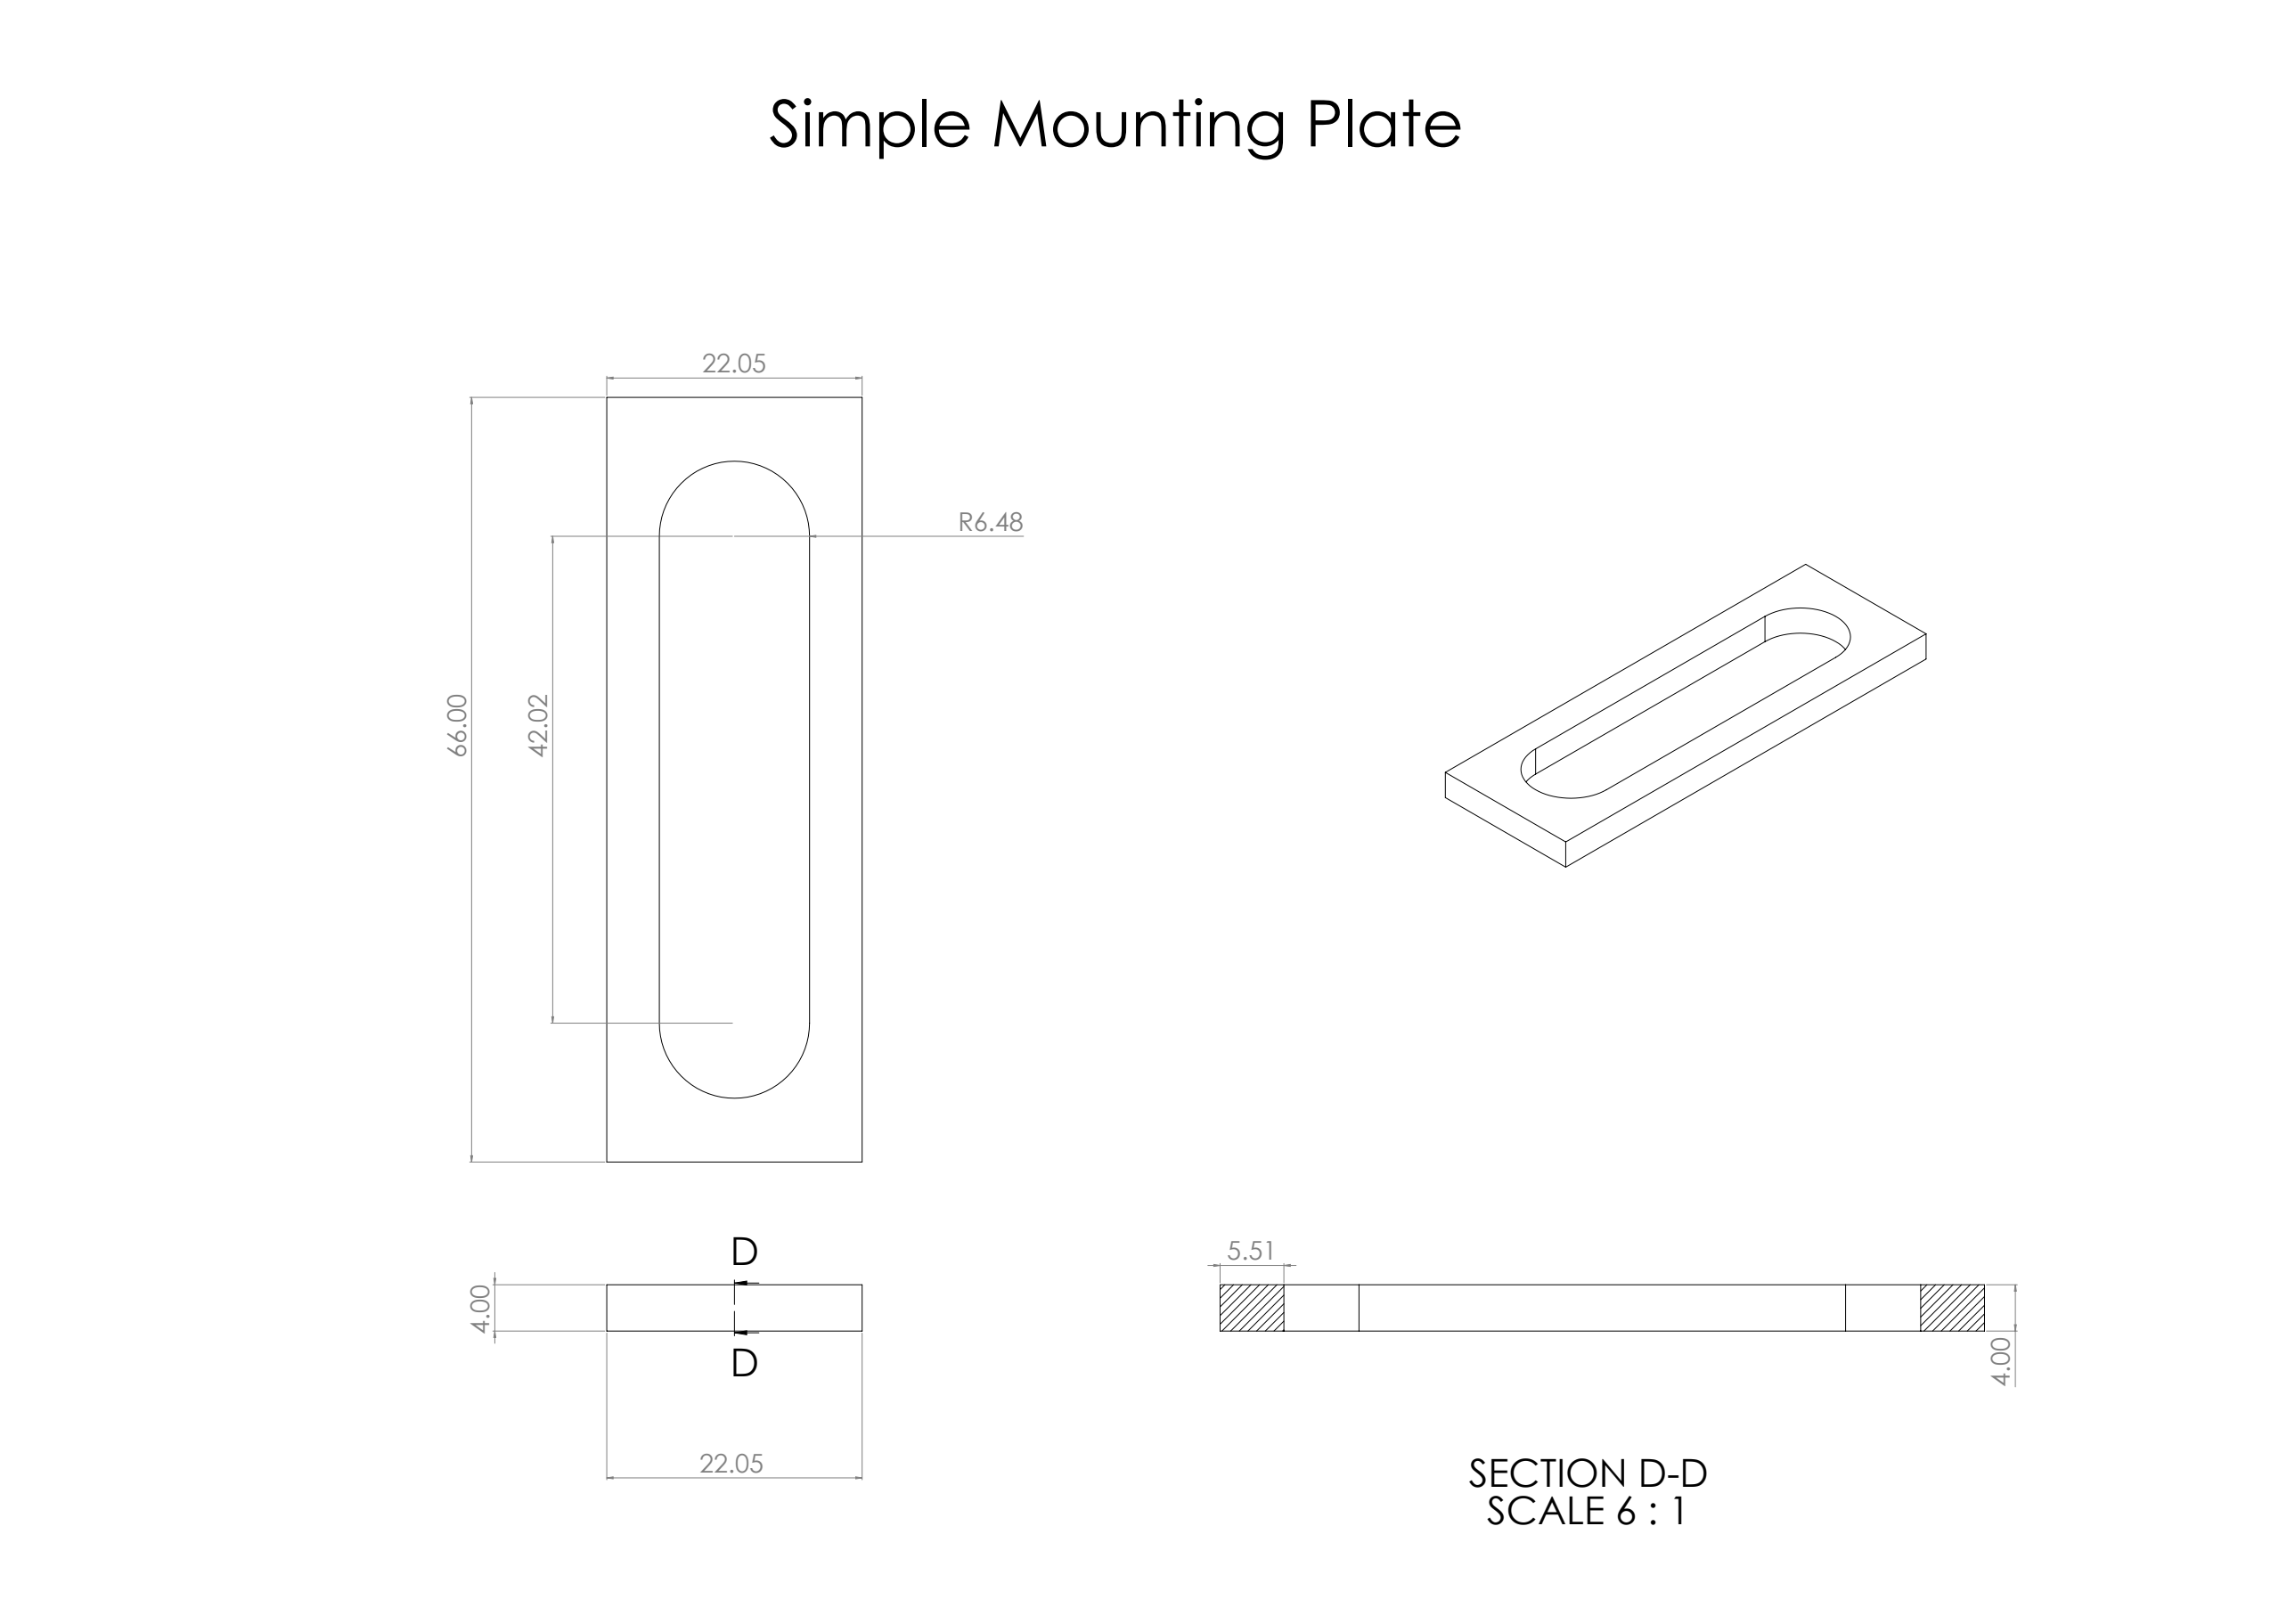
ISO-10303-21;
HEADER;
FILE_DESCRIPTION (('STEP AP214'),
    '1' );
FILE_NAME ('Simple Mounting Plate.step',
    '2026-10-24T21:31:31',
    ( '' ),
    ( '' ),
    'SwSTEP 2.0',
    'SolidWorks 2025',
    '' );
FILE_SCHEMA (( 'AUTOMOTIVE_DESIGN' ));
ENDSEC;

DATA;
#29=DIRECTION ( 'NONE',  ( 1.000000000000000000, 0.000000000000000000, 0.000000000000000000 ) ) ;
#109=DIRECTION ( 'NONE',  ( 0.000000000000000000, 1.000000000000000000, 0.000000000000000000 ) ) ;
#168=( NAMED_UNIT ( * ) PLANE_ANGLE_UNIT ( ) SI_UNIT ( $, .RADIAN. ) );
#183=CIRCLE ( 'NONE', #7797, 6.484807146443463566 ) ;
#379=LINE ( 'NONE', #14467, #12326 ) ;
#390=FACE_OUTER_BOUND ( 'NONE', #10750, .T. ) ;
#422=ORIENTED_EDGE ( 'NONE', *, *, #2866, .F. ) ;
#457=CARTESIAN_POINT ( 'NONE',  ( 80.18290120114222930, 29.52935533987996664, -21.00807340887166674 ) ) ;
#476=EDGE_CURVE ( 'NONE', #7436, #10628, #11850, .T. ) ;
#568=CIRCLE ( 'NONE', #806, 6.484807146443463566 ) ;
#583=FACE_OUTER_BOUND ( 'NONE', #10613, .T. ) ;
#609=EDGE_CURVE ( 'NONE', #7436, #1277, #1384, .T. ) ;
#623=( LENGTH_UNIT ( ) NAMED_UNIT ( * ) SI_UNIT ( .MILLI., .METRE. ) );
#791=VERTEX_POINT ( 'NONE', #9257 ) ;
#806=AXIS2_PLACEMENT_3D ( 'NONE', #12943, #2078, #13935 ) ;
#820=EDGE_LOOP ( 'NONE', ( #5722, #8057, #10459, #9791, #8309 ) ) ;
#827=CARTESIAN_POINT ( 'NONE',  ( 80.18290120114222930, 29.52935533987996664, 21.00807340887166674 ) ) ;
#863=CARTESIAN_POINT ( 'NONE',  ( 67.21328690825529861, 29.52935533987996664, -21.00807340887166674 ) ) ;
#928=AXIS2_PLACEMENT_3D ( 'NONE', #14541, #7614, #1981 ) ;
#984=DIRECTION ( 'NONE',  ( 0.000000000000000000, 0.000000000000000000, 1.000000000000000000 ) ) ;
#1030=AXIS2_PLACEMENT_3D ( 'NONE', #11882, #5895, #6042 ) ;
#1049=ORIENTED_EDGE ( 'NONE', *, *, #13035, .F. ) ;
#1079=DIRECTION ( 'NONE',  ( 0.000000000000000000, 0.000000000000000000, 1.000000000000000000 ) ) ;
#1080=ORIENTED_EDGE ( 'NONE', *, *, #1195, .F. ) ;
#1195=EDGE_CURVE ( 'NONE', #10628, #10836, #7216, .T. ) ;
#1277=VERTEX_POINT ( 'NONE', #3964 ) ;
#1327=AXIS2_PLACEMENT_3D ( 'NONE', #8905, #1894, #6592 ) ;
#1376=LINE ( 'NONE', #7228, #11447 ) ;
#1384=LINE ( 'NONE', #457, #2184 ) ;
#1482=CARTESIAN_POINT ( 'NONE',  ( 0.000000000000000000, 25.52935533987996664, 0.000000000000000000 ) ) ;
#1489=ORIENTED_EDGE ( 'NONE', *, *, #10313, .T. ) ;
#1494=DIRECTION ( 'NONE',  ( 0.000000000000000000, 0.000000000000000000, 1.000000000000000000 ) ) ;
#1505=UNCERTAINTY_MEASURE_WITH_UNIT (LENGTH_MEASURE( 1.000000000000000082E-05 ), #623, 'distance_accuracy_value', 'NONE');
#1520=DIRECTION ( 'NONE',  ( -0.000000000000000000, -0.000000000000000000, -1.000000000000000000 ) ) ;
#1550=ORIENTED_EDGE ( 'NONE', *, *, #14612, .F. ) ;
#1557=SHAPE_REPRESENTATION ( 'Simple Mounting Plate', ( #6315 ), #10740 ) ;
#1651=UNCERTAINTY_MEASURE_WITH_UNIT (LENGTH_MEASURE( 1.000000000000000082E-05 ), #7097, 'distance_accuracy_value', 'NONE');
#1684=DIRECTION ( 'NONE',  ( -1.000000000000000000, -0.000000000000000000, -0.000000000000000000 ) ) ;
#1734=DIRECTION ( 'NONE',  ( 1.000000000000000000, 0.000000000000000000, 0.000000000000000000 ) ) ;
#1764=VECTOR ( 'NONE', #15120, 1000.000000000000000 ) ;
#1873=ADVANCED_FACE ( 'NONE', ( #10648, #14344 ), #12017, .F. ) ;
#1894=DIRECTION ( 'NONE',  ( -1.000000000000000000, 0.000000000000000000, 0.000000000000000000 ) ) ;
#1912=ORIENTED_EDGE ( 'NONE', *, *, #2866, .T. ) ;
#1981=DIRECTION ( 'NONE',  ( 0.000000000000000000, 0.000000000000000000, -1.000000000000000000 ) ) ;
#2036=EDGE_CURVE ( 'NONE', #12382, #4409, #3728, .T. ) ;
#2078=DIRECTION ( 'NONE',  ( 0.000000000000000000, 1.000000000000000000, 0.000000000000000000 ) ) ;
#2087=SHAPE_REPRESENTATION_RELATIONSHIP ( 'NONE' , 'NONE' ,  #1557, #14388 ) ;
#2104=CYLINDRICAL_SURFACE ( 'NONE', #3264, 6.484807146443463566 ) ;
#2154=CLOSED_SHELL ( 'NONE', ( #8223, #12212, #1873, #6816, #3020, #5563, #3592, #7389, #14535, #15006, #9629 ) ) ;
#2184=VECTOR ( 'NONE', #14243, 1000.000000000000000 ) ;
#2233=DIRECTION ( 'NONE',  ( -0.000000000000000000, -1.000000000000000000, -0.000000000000000000 ) ) ;
#2372=ORIENTED_EDGE ( 'NONE', *, *, #14612, .T. ) ;
#2603=CARTESIAN_POINT ( 'NONE',  ( 62.67308791069655882, 25.52935533987996664, -33.00000000000013500 ) ) ;
#2662=ORIENTED_EDGE ( 'NONE', *, *, #6455, .F. ) ;
#2724=VECTOR ( 'NONE', #7198, 1000.000000000000000 ) ;
#2775=AXIS2_PLACEMENT_3D ( 'NONE', #14477, #3923, #8618 ) ;
#2819=PLANE ( 'NONE',  #15180 ) ;
#2866=EDGE_CURVE ( 'NONE', #3904, #14153, #13128, .T. ) ;
#2949=CARTESIAN_POINT ( 'NONE',  ( 73.69809405469877106, 29.52935533987996664, -21.00807340887166674 ) ) ;
#2992=ORIENTED_EDGE ( 'NONE', *, *, #10935, .F. ) ;
#3020=ADVANCED_FACE ( 'NONE', ( #5114 ), #11033, .F. ) ;
#3026=CARTESIAN_POINT ( 'NONE',  ( 80.18290120114222930, 25.52935533987996664, 21.00807340887166674 ) ) ;
#3032=DIRECTION ( 'NONE',  ( 0.000000000000000000, 0.000000000000000000, -1.000000000000000000 ) ) ;
#3108=CARTESIAN_POINT ( 'NONE',  ( 62.67308791069655882, 29.52935533987996664, 33.00000000000014211 ) ) ;
#3186=DIRECTION ( 'NONE',  ( 0.000000000000000000, 0.000000000000000000, 1.000000000000000000 ) ) ;
#3189=EDGE_CURVE ( 'NONE', #14936, #3904, #9655, .T. ) ;
#3207=FACE_OUTER_BOUND ( 'NONE', #4528, .T. ) ;
#3235=PLANE ( 'NONE',  #15227 ) ;
#3263=DIRECTION ( 'NONE',  ( -0.000000000000000000, -1.000000000000000000, -0.000000000000000000 ) ) ;
#3264=AXIS2_PLACEMENT_3D ( 'NONE', #6802, #13886, #3340 ) ;
#3284=ORIENTED_EDGE ( 'NONE', *, *, #5084, .F. ) ;
#3339=ORIENTED_EDGE ( 'NONE', *, *, #10313, .F. ) ;
#3340=DIRECTION ( 'NONE',  ( 0.000000000000000000, 0.000000000000000000, -1.000000000000000000 ) ) ;
#3384=FACE_OUTER_BOUND ( 'NONE', #10476, .T. ) ;
#3387=VECTOR ( 'NONE', #8666, 1000.000000000000000 ) ;
#3517=PRODUCT_DEFINITION_CONTEXT ( 'detailed design', #5959, 'design' ) ;
#3592=ADVANCED_FACE ( 'NONE', ( #10240 ), #3235, .F. ) ;
#3719=CARTESIAN_POINT ( 'NONE',  ( 84.72310019870096198, 29.52935533987996664, -33.00000000000013500 ) ) ;
#3728=LINE ( 'NONE', #14048, #4112 ) ;
#3738=VERTEX_POINT ( 'NONE', #6599 ) ;
#3748=CARTESIAN_POINT ( 'NONE',  ( 80.18290120114222930, 25.52935533987996664, -21.00807340887166674 ) ) ;
#3796=CARTESIAN_POINT ( 'NONE',  ( 80.18290120114222930, 29.52935533987996664, -21.00807340887166674 ) ) ;
#3904=VERTEX_POINT ( 'NONE', #5267 ) ;
#3923=DIRECTION ( 'NONE',  ( 1.000000000000000000, 0.000000000000000000, 0.000000000000000000 ) ) ;
#3946=DIRECTION ( 'NONE',  ( -1.000000000000000000, 0.000000000000000000, -0.000000000000000000 ) ) ;
#3964=CARTESIAN_POINT ( 'NONE',  ( 80.18290120114222930, 29.52935533987996664, -21.00807340887166674 ) ) ;
#3989=DIRECTION ( 'NONE',  ( -0.000000000000000000, -0.000000000000000000, -1.000000000000000000 ) ) ;
#4000=EDGE_CURVE ( 'NONE', #11210, #8448, #4643, .T. ) ;
#4022=ORIENTED_EDGE ( 'NONE', *, *, #7061, .T. ) ;
#4082=CARTESIAN_POINT ( 'NONE',  ( 0.000000000000000000, 0.000000000000000000, 0.000000000000000000 ) ) ;
#4112=VECTOR ( 'NONE', #10512, 1000.000000000000000 ) ;
#4123=ORIENTED_EDGE ( 'NONE', *, *, #5084, .T. ) ;
#4172=VERTEX_POINT ( 'NONE', #15048 ) ;
#4217=CIRCLE ( 'NONE', #1030, 6.484807146443463566 ) ;
#4250=VERTEX_POINT ( 'NONE', #6048 ) ;
#4296=CARTESIAN_POINT ( 'NONE',  ( 0.000000000000000000, 29.52935533987996664, 0.000000000000000000 ) ) ;
#4311=AXIS2_PLACEMENT_3D ( 'NONE', #4296, #4456, #8001 ) ;
#4409=VERTEX_POINT ( 'NONE', #7856 ) ;
#4443=VERTEX_POINT ( 'NONE', #10395 ) ;
#4456=DIRECTION ( 'NONE',  ( 0.000000000000000000, 1.000000000000000000, 0.000000000000000000 ) ) ;
#4528=EDGE_LOOP ( 'NONE', ( #11682, #1049, #9936, #1912 ) ) ;
#4547=EDGE_LOOP ( 'NONE', ( #14272, #13147, #6987, #3284 ) ) ;
#4643=LINE ( 'NONE', #863, #6660 ) ;
#4668=AXIS2_PLACEMENT_3D ( 'NONE', #14874, #3263, #5740 ) ;
#4759=VECTOR ( 'NONE', #3989, 1000.000000000000000 ) ;
#4773=DIRECTION ( 'NONE',  ( 0.000000000000000000, 0.000000000000000000, 1.000000000000000000 ) ) ;
#4825=AXIS2_PLACEMENT_3D ( 'NONE', #8741, #9919, #12290 ) ;
#4891=CARTESIAN_POINT ( 'NONE',  ( 84.72310019870096198, 29.52935533987996664, 33.00000000000014211 ) ) ;
#4982=VECTOR ( 'NONE', #12387, 1000.000000000000000 ) ;
#4984=CIRCLE ( 'NONE', #13574, 6.484807146443463566 ) ;
#4992=ORIENTED_EDGE ( 'NONE', *, *, #11137, .T. ) ;
#5036=CARTESIAN_POINT ( 'NONE',  ( 73.69809405469877106, 25.52935533987996664, -21.00807340887166674 ) ) ;
#5084=EDGE_CURVE ( 'NONE', #4409, #8448, #4984, .T. ) ;
#5086=PLANE ( 'NONE',  #2775 ) ;
#5114=FACE_OUTER_BOUND ( 'NONE', #5541, .T. ) ;
#5236=ORIENTED_EDGE ( 'NONE', *, *, #13202, .T. ) ;
#5267=CARTESIAN_POINT ( 'NONE',  ( 84.72310019870096198, 29.52935533987996664, 33.00000000000014211 ) ) ;
#5357=CARTESIAN_POINT ( 'NONE',  ( 67.21328690825529861, 29.52935533987996664, 21.00807340887166674 ) ) ;
#5366=PLANE ( 'NONE',  #4825 ) ;
#5406=DIRECTION ( 'NONE',  ( 0.000000000000000000, 0.000000000000000000, 1.000000000000000000 ) ) ;
#5434=EDGE_LOOP ( 'NONE', ( #2992, #12627, #6836, #9824 ) ) ;
#5439=ORIENTED_EDGE ( 'NONE', *, *, #2036, .T. ) ;
#5518=LINE ( 'NONE', #10203, #10026 ) ;
#5541=EDGE_LOOP ( 'NONE', ( #9090, #422, #8691, #6135 ) ) ;
#5563=ADVANCED_FACE ( 'NONE', ( #3207 ), #12439, .F. ) ;
#5573=FACE_OUTER_BOUND ( 'NONE', #8073, .T. ) ;
#5580=CARTESIAN_POINT ( 'NONE',  ( 67.21328690825529861, 25.52935533987996664, -21.00807340887166674 ) ) ;
#5616=ORIENTED_EDGE ( 'NONE', *, *, #12795, .F. ) ;
#5660=VERTEX_POINT ( 'NONE', #5682 ) ;
#5682=CARTESIAN_POINT ( 'NONE',  ( 67.21328690825529861, 25.52935533987996664, 21.00807340887166674 ) ) ;
#5722=ORIENTED_EDGE ( 'NONE', *, *, #11137, .F. ) ;
#5740=DIRECTION ( 'NONE',  ( 0.000000000000000000, 0.000000000000000000, -1.000000000000000000 ) ) ;
#5748=LINE ( 'NONE', #5580, #11967 ) ;
#5762=ORIENTED_EDGE ( 'NONE', *, *, #12795, .T. ) ;
#5829=ORIENTED_EDGE ( 'NONE', *, *, #11146, .F. ) ;
#5852=DIRECTION ( 'NONE',  ( 0.000000000000000000, 0.000000000000000000, 1.000000000000000000 ) ) ;
#5895=DIRECTION ( 'NONE',  ( 0.000000000000000000, 1.000000000000000000, 0.000000000000000000 ) ) ;
#5959=APPLICATION_CONTEXT ( 'automotive_design' ) ;
#5992=EDGE_LOOP ( 'NONE', ( #6152, #11893, #2662, #5829 ) ) ;
#6042=DIRECTION ( 'NONE',  ( 0.000000000000000000, 0.000000000000000000, 1.000000000000000000 ) ) ;
#6048=CARTESIAN_POINT ( 'NONE',  ( 62.67308791069655882, 25.52935533987996664, 33.00000000000014211 ) ) ;
#6063=ORIENTED_EDGE ( 'NONE', *, *, #6904, .T. ) ;
#6122=DIRECTION ( 'NONE',  ( 0.000000000000000000, 1.000000000000000000, 0.000000000000000000 ) ) ;
#6135=ORIENTED_EDGE ( 'NONE', *, *, #7055, .T. ) ;
#6147=EDGE_CURVE ( 'NONE', #12382, #11210, #568, .T. ) ;
#6152=ORIENTED_EDGE ( 'NONE', *, *, #13269, .F. ) ;
#6179=FACE_OUTER_BOUND ( 'NONE', #9104, .T. ) ;
#6315=AXIS2_PLACEMENT_3D ( 'NONE', #4082, #8567, #11096 ) ;
#6455=EDGE_CURVE ( 'NONE', #14153, #4443, #11150, .T. ) ;
#6566=CIRCLE ( 'NONE', #10757, 6.484807146443463566 ) ;
#6570=ORIENTED_EDGE ( 'NONE', *, *, #10935, .T. ) ;
#6592=DIRECTION ( 'NONE',  ( 0.000000000000000000, 0.000000000000000000, 1.000000000000000000 ) ) ;
#6599=CARTESIAN_POINT ( 'NONE',  ( 62.67308791069655882, 29.52935533987996664, -33.00000000000013500 ) ) ;
#6660=VECTOR ( 'NONE', #13958, 1000.000000000000000 ) ;
#6788=VECTOR ( 'NONE', #4773, 1000.000000000000000 ) ;
#6802=CARTESIAN_POINT ( 'NONE',  ( 73.69809405469877106, 29.52935533987996664, 21.00807340887166674 ) ) ;
#6816=ADVANCED_FACE ( 'NONE', ( #583 ), #2819, .F. ) ;
#6836=ORIENTED_EDGE ( 'NONE', *, *, #13014, .T. ) ;
#6839=VERTEX_POINT ( 'NONE', #5357 ) ;
#6847=VECTOR ( 'NONE', #2233, 1000.000000000000000 ) ;
#6878=CARTESIAN_POINT ( 'NONE',  ( 62.67308791069655882, 29.52935533987996664, -33.00000000000013500 ) ) ;
#6904=EDGE_CURVE ( 'NONE', #3904, #4172, #12138, .T. ) ;
#6936=VECTOR ( 'NONE', #10460, 1000.000000000000000 ) ;
#6987=ORIENTED_EDGE ( 'NONE', *, *, #4000, .T. ) ;
#7039=STYLED_ITEM('',(#15258),#9491);
#7055=EDGE_CURVE ( 'NONE', #14936, #4250, #10357, .T. ) ;
#7061=EDGE_CURVE ( 'NONE', #6839, #5660, #5518, .T. ) ;
#7081=DIRECTION ( 'NONE',  ( 1.000000000000000000, 0.000000000000000000, 0.000000000000000000 ) ) ;
#7097=( LENGTH_UNIT ( ) NAMED_UNIT ( * ) SI_UNIT ( .MILLI., .METRE. ) );
#7198=DIRECTION ( 'NONE',  ( -0.000000000000000000, -1.000000000000000000, -0.000000000000000000 ) ) ;
#7216=LINE ( 'NONE', #3748, #7940 ) ;
#7228=CARTESIAN_POINT ( 'NONE',  ( 62.67308791069655882, 25.52935533987996664, 33.00000000000014211 ) ) ;
#7279=ORIENTED_EDGE ( 'NONE', *, *, #10225, .F. ) ;
#7320=ORIENTED_EDGE ( 'NONE', *, *, #609, .T. ) ;
#7389=ADVANCED_FACE ( 'NONE', ( #8834 ), #13685, .F. ) ;
#7436=VERTEX_POINT ( 'NONE', #827 ) ;
#7614=DIRECTION ( 'NONE',  ( -0.000000000000000000, -1.000000000000000000, -0.000000000000000000 ) ) ;
#7698=CARTESIAN_POINT ( 'NONE',  ( 62.67308791069655882, 29.52935533987996664, -33.00000000000013500 ) ) ;
#7718=( NAMED_UNIT ( * ) SI_UNIT ( $, .STERADIAN. ) SOLID_ANGLE_UNIT ( ) );
#7735=FACE_OUTER_BOUND ( 'NONE', #5434, .T. ) ;
#7763=CARTESIAN_POINT ( 'NONE',  ( 84.72310019870096198, 25.52935533987996664, -33.00000000000013500 ) ) ;
#7797=AXIS2_PLACEMENT_3D ( 'NONE', #5036, #6122, #1494 ) ;
#7804=CYLINDRICAL_SURFACE ( 'NONE', #4668, 6.484807146443463566 ) ;
#7856=CARTESIAN_POINT ( 'NONE',  ( 73.69809405469877106, 25.52935533987996664, -27.49288055531513209 ) ) ;
#7940=VECTOR ( 'NONE', #1520, 1000.000000000000000 ) ;
#8001=DIRECTION ( 'NONE',  ( 0.000000000000000000, -0.000000000000000000, 1.000000000000000000 ) ) ;
#8057=ORIENTED_EDGE ( 'NONE', *, *, #6147, .F. ) ;
#8073=EDGE_LOOP ( 'NONE', ( #13422, #5439, #3339, #13303 ) ) ;
#8223=ADVANCED_FACE ( 'NONE', ( #5573 ), #7804, .F. ) ;
#8309=ORIENTED_EDGE ( 'NONE', *, *, #13014, .F. ) ;
#8370=ORIENTED_EDGE ( 'NONE', *, *, #4000, .F. ) ;
#8386=AXIS2_PLACEMENT_3D ( 'NONE', #9960, #3032, #3946 ) ;
#8413=CARTESIAN_POINT ( 'NONE',  ( 80.18290120114222930, 25.52935533987996664, -21.00807340887166674 ) ) ;
#8448=VERTEX_POINT ( 'NONE', #13116 ) ;
#8467=LINE ( 'NONE', #2603, #13061 ) ;
#8567=DIRECTION ( 'NONE',  ( 0.000000000000000000, 0.000000000000000000, 1.000000000000000000 ) ) ;
#8618=DIRECTION ( 'NONE',  ( 0.000000000000000000, 0.000000000000000000, -1.000000000000000000 ) ) ;
#8666=DIRECTION ( 'NONE',  ( -0.000000000000000000, -0.000000000000000000, -1.000000000000000000 ) ) ;
#8691=ORIENTED_EDGE ( 'NONE', *, *, #3189, .F. ) ;
#8696=DIRECTION ( 'NONE',  ( 0.000000000000000000, 0.000000000000000000, 1.000000000000000000 ) ) ;
#8741=CARTESIAN_POINT ( 'NONE',  ( 80.18290120114222930, 29.52935533987996664, -21.00807340887166674 ) ) ;
#8764=CARTESIAN_POINT ( 'NONE',  ( 73.69809405469877106, 25.52935533987996664, 21.00807340887166674 ) ) ;
#8834=FACE_OUTER_BOUND ( 'NONE', #4547, .T. ) ;
#8905=CARTESIAN_POINT ( 'NONE',  ( 84.72310019870096198, 29.52935533987996664, -33.00000000000013500 ) ) ;
#9090=ORIENTED_EDGE ( 'NONE', *, *, #11146, .T. ) ;
#9104=EDGE_LOOP ( 'NONE', ( #1080, #13615, #7320, #11727 ) ) ;
#9257=CARTESIAN_POINT ( 'NONE',  ( 62.67308791069655882, 25.52935533987996664, -33.00000000000013500 ) ) ;
#9292=LINE ( 'NONE', #7698, #4982 ) ;
#9388=LINE ( 'NONE', #13076, #14327 ) ;
#9491=MANIFOLD_SOLID_BREP ( 'Boss-Extrude18', #2154 ) ;
#9552=LINE ( 'NONE', #14084, #6788 ) ;
#9579=CARTESIAN_POINT ( 'NONE',  ( 62.67308791069655882, 29.52935533987996664, 33.00000000000014211 ) ) ;
#9625=CARTESIAN_POINT ( 'NONE',  ( 67.21328690825529861, 29.52935533987996664, -21.00807340887166674 ) ) ;
#9629=ADVANCED_FACE ( 'NONE', ( #6179 ), #5366, .T. ) ;
#9630=CARTESIAN_POINT ( 'NONE',  ( 73.69809405469877106, 29.52935533987996664, -27.49288055531513209 ) ) ;
#9655=LINE ( 'NONE', #9579, #10802 ) ;
#9656=VECTOR ( 'NONE', #10658, 1000.000000000000000 ) ;
#9664=CARTESIAN_POINT ( 'NONE',  ( 84.72310019870096198, 25.52935533987996664, 33.00000000000014211 ) ) ;
#9791=ORIENTED_EDGE ( 'NONE', *, *, #609, .F. ) ;
#9824=ORIENTED_EDGE ( 'NONE', *, *, #476, .T. ) ;
#9909=CARTESIAN_POINT ( 'NONE',  ( 62.67308791069655882, 29.52935533987996664, -33.00000000000013500 ) ) ;
#9919=DIRECTION ( 'NONE',  ( -1.000000000000000000, 0.000000000000000000, 0.000000000000000000 ) ) ;
#9936=ORIENTED_EDGE ( 'NONE', *, *, #6904, .F. ) ;
#9960=CARTESIAN_POINT ( 'NONE',  ( 62.67308791069655882, 29.52935533987996664, 33.00000000000014211 ) ) ;
#9963=ORIENTED_EDGE ( 'NONE', *, *, #13035, .T. ) ;
#10026=VECTOR ( 'NONE', #14889, 1000.000000000000000 ) ;
#10155=PRODUCT ( 'Simple Mounting Plate', 'Simple Mounting Plate', '', ( #12240 ) ) ;
#10203=CARTESIAN_POINT ( 'NONE',  ( 67.21328690825529861, 29.52935533987996664, 21.00807340887166674 ) ) ;
#10225=EDGE_CURVE ( 'NONE', #8448, #5660, #5748, .T. ) ;
#10240=FACE_OUTER_BOUND ( 'NONE', #10409, .T. ) ;
#10272=LINE ( 'NONE', #6878, #1764 ) ;
#10312=FACE_BOUND ( 'NONE', #820, .T. ) ;
#10313=EDGE_CURVE ( 'NONE', #10836, #4409, #183, .T. ) ;
#10329=( NAMED_UNIT ( * ) PLANE_ANGLE_UNIT ( ) SI_UNIT ( $, .RADIAN. ) );
#10357=LINE ( 'NONE', #12510, #12733 ) ;
#10395=CARTESIAN_POINT ( 'NONE',  ( 84.72310019870096198, 25.52935533987996664, -33.00000000000013500 ) ) ;
#10409=EDGE_LOOP ( 'NONE', ( #13917, #1550, #11772, #9963 ) ) ;
#10459=ORIENTED_EDGE ( 'NONE', *, *, #10584, .F. ) ;
#10460=DIRECTION ( 'NONE',  ( -0.000000000000000000, -1.000000000000000000, -0.000000000000000000 ) ) ;
#10476=EDGE_LOOP ( 'NONE', ( #5762, #13529, #6063, #5236 ) ) ;
#10512=DIRECTION ( 'NONE',  ( -0.000000000000000000, -1.000000000000000000, -0.000000000000000000 ) ) ;
#10533=DIRECTION ( 'NONE',  ( 0.000000000000000000, -0.000000000000000000, 1.000000000000000000 ) ) ;
#10584=EDGE_CURVE ( 'NONE', #1277, #12382, #12221, .T. ) ;
#10613=EDGE_LOOP ( 'NONE', ( #11963, #13071, #5616, #2372 ) ) ;
#10628=VERTEX_POINT ( 'NONE', #3026 ) ;
#10648=FACE_OUTER_BOUND ( 'NONE', #5992, .T. ) ;
#10658=DIRECTION ( 'NONE',  ( -0.000000000000000000, -1.000000000000000000, -0.000000000000000000 ) ) ;
#10711=( NAMED_UNIT ( * ) SI_UNIT ( $, .STERADIAN. ) SOLID_ANGLE_UNIT ( ) );
#10740=( GEOMETRIC_REPRESENTATION_CONTEXT ( 3 ) GLOBAL_UNCERTAINTY_ASSIGNED_CONTEXT ( ( #1505 ) ) GLOBAL_UNIT_ASSIGNED_CONTEXT ( ( #623, #10329, #7718 ) ) REPRESENTATION_CONTEXT ( 'NONE', 'WORKASPACE' ) );
#10750=EDGE_LOOP ( 'NONE', ( #7279, #8370, #4992, #4022 ) ) ;
#10757=AXIS2_PLACEMENT_3D ( 'NONE', #8764, #13322, #8696 ) ;
#10791=SHAPE_DEFINITION_REPRESENTATION ( #12488, #1557 ) ;
#10802=VECTOR ( 'NONE', #29, 1000.000000000000000 ) ;
#10836=VERTEX_POINT ( 'NONE', #8413 ) ;
#10935=EDGE_CURVE ( 'NONE', #5660, #10628, #6566, .T. ) ;
#10956=ORIENTED_EDGE ( 'NONE', *, *, #10225, .T. ) ;
#11033=PLANE ( 'NONE',  #8386 ) ;
#11096=DIRECTION ( 'NONE',  ( 1.000000000000000000, 0.000000000000000000, 0.000000000000000000 ) ) ;
#11137=EDGE_CURVE ( 'NONE', #11210, #6839, #9552, .T. ) ;
#11146=EDGE_CURVE ( 'NONE', #4250, #14153, #1376, .T. ) ;
#11150=LINE ( 'NONE', #7763, #4759 ) ;
#11210=VERTEX_POINT ( 'NONE', #9625 ) ;
#11246=DIRECTION ( 'NONE',  ( 0.000000000000000000, 1.000000000000000000, 0.000000000000000000 ) ) ;
#11379=PLANE ( 'NONE',  #4311 ) ;
#11417=DIRECTION ( 'NONE',  ( -0.000000000000000000, -1.000000000000000000, -0.000000000000000000 ) ) ;
#11447=VECTOR ( 'NONE', #7081, 1000.000000000000000 ) ;
#11475=AXIS2_PLACEMENT_3D ( 'NONE', #2949, #11246, #5406 ) ;
#11682=ORIENTED_EDGE ( 'NONE', *, *, #6455, .T. ) ;
#11685=DIRECTION ( 'NONE',  ( -1.000000000000000000, -0.000000000000000000, -0.000000000000000000 ) ) ;
#11706=MECHANICAL_DESIGN_GEOMETRIC_PRESENTATION_REPRESENTATION('',(#7039),#13915);
#11727=ORIENTED_EDGE ( 'NONE', *, *, #12947, .T. ) ;
#11772=ORIENTED_EDGE ( 'NONE', *, *, #13202, .F. ) ;
#11774=CARTESIAN_POINT ( 'NONE',  ( 80.18290120114222930, 29.52935533987996664, 21.00807340887166674 ) ) ;
#11850=LINE ( 'NONE', #11774, #6847 ) ;
#11882=CARTESIAN_POINT ( 'NONE',  ( 73.69809405469877106, 29.52935533987996664, 21.00807340887166674 ) ) ;
#11893=ORIENTED_EDGE ( 'NONE', *, *, #12483, .F. ) ;
#11914=EDGE_LOOP ( 'NONE', ( #1489, #4123, #10956, #6570, #14624 ) ) ;
#11963=ORIENTED_EDGE ( 'NONE', *, *, #13269, .T. ) ;
#11967=VECTOR ( 'NONE', #3186, 1000.000000000000000 ) ;
#12017=PLANE ( 'NONE',  #15196 ) ;
#12138=LINE ( 'NONE', #12429, #3387 ) ;
#12212=ADVANCED_FACE ( 'NONE', ( #3384, #10312 ), #11379, .T. ) ;
#12215=PRODUCT_DEFINITION_FORMATION_WITH_SPECIFIED_SOURCE ( 'ANY', '', #10155, .NOT_KNOWN. ) ;
#12221=CIRCLE ( 'NONE', #11475, 6.484807146443463566 ) ;
#12240=PRODUCT_CONTEXT ( 'NONE', #14245, 'mechanical' ) ;
#12290=DIRECTION ( 'NONE',  ( 0.000000000000000000, 0.000000000000000000, 1.000000000000000000 ) ) ;
#12292=PRODUCT_DEFINITION ( 'UNKNOWN', '', #12215, #3517 ) ;
#12326=VECTOR ( 'NONE', #1684, 1000.000000000000000 ) ;
#12382=VERTEX_POINT ( 'NONE', #9630 ) ;
#12387=DIRECTION ( 'NONE',  ( -0.000000000000000000, -1.000000000000000000, -0.000000000000000000 ) ) ;
#12429=CARTESIAN_POINT ( 'NONE',  ( 84.72310019870096198, 29.52935533987996664, -33.00000000000013500 ) ) ;
#12439=PLANE ( 'NONE',  #1327 ) ;
#12483=EDGE_CURVE ( 'NONE', #4443, #791, #379, .T. ) ;
#12488=PRODUCT_DEFINITION_SHAPE ( 'NONE', 'NONE',  #12292 ) ;
#12510=CARTESIAN_POINT ( 'NONE',  ( 62.67308791069655882, 29.52935533987996664, 33.00000000000014211 ) ) ;
#12627=ORIENTED_EDGE ( 'NONE', *, *, #7061, .F. ) ;
#12631=CARTESIAN_POINT ( 'NONE',  ( 62.67308791069655882, 29.52935533987996664, -33.00000000000013500 ) ) ;
#12733=VECTOR ( 'NONE', #11417, 1000.000000000000000 ) ;
#12795=EDGE_CURVE ( 'NONE', #3738, #14936, #10272, .T. ) ;
#12943=CARTESIAN_POINT ( 'NONE',  ( 73.69809405469877106, 29.52935533987996664, -21.00807340887166674 ) ) ;
#12947=EDGE_CURVE ( 'NONE', #1277, #10836, #14352, .T. ) ;
#13014=EDGE_CURVE ( 'NONE', #6839, #7436, #4217, .T. ) ;
#13035=EDGE_CURVE ( 'NONE', #4172, #4443, #14271, .T. ) ;
#13061=VECTOR ( 'NONE', #5852, 1000.000000000000000 ) ;
#13071=ORIENTED_EDGE ( 'NONE', *, *, #7055, .F. ) ;
#13076=CARTESIAN_POINT ( 'NONE',  ( 62.67308791069655882, 29.52935533987996664, -33.00000000000013500 ) ) ;
#13116=CARTESIAN_POINT ( 'NONE',  ( 67.21328690825529861, 25.52935533987996664, -21.00807340887166674 ) ) ;
#13128=LINE ( 'NONE', #4891, #2724 ) ;
#13147=ORIENTED_EDGE ( 'NONE', *, *, #6147, .T. ) ;
#13202=EDGE_CURVE ( 'NONE', #4172, #3738, #9388, .T. ) ;
#13269=EDGE_CURVE ( 'NONE', #791, #4250, #8467, .T. ) ;
#13303=ORIENTED_EDGE ( 'NONE', *, *, #12947, .F. ) ;
#13322=DIRECTION ( 'NONE',  ( 0.000000000000000000, 1.000000000000000000, 0.000000000000000000 ) ) ;
#13422=ORIENTED_EDGE ( 'NONE', *, *, #10584, .T. ) ;
#13509=DIRECTION ( 'NONE',  ( 0.000000000000000000, 0.000000000000000000, -1.000000000000000000 ) ) ;
#13529=ORIENTED_EDGE ( 'NONE', *, *, #3189, .T. ) ;
#13574=AXIS2_PLACEMENT_3D ( 'NONE', #15088, #15003, #984 ) ;
#13615=ORIENTED_EDGE ( 'NONE', *, *, #476, .F. ) ;
#13685=CYLINDRICAL_SURFACE ( 'NONE', #928, 6.484807146443463566 ) ;
#13886=DIRECTION ( 'NONE',  ( -0.000000000000000000, -1.000000000000000000, -0.000000000000000000 ) ) ;
#13915=( GEOMETRIC_REPRESENTATION_CONTEXT ( 3 ) GLOBAL_UNCERTAINTY_ASSIGNED_CONTEXT ( ( #1651 ) ) GLOBAL_UNIT_ASSIGNED_CONTEXT ( ( #7097, #168, #10711 ) ) REPRESENTATION_CONTEXT ( 'NONE', 'WORKASPACE' ) );
#13917=ORIENTED_EDGE ( 'NONE', *, *, #12483, .T. ) ;
#13935=DIRECTION ( 'NONE',  ( 0.000000000000000000, 0.000000000000000000, 1.000000000000000000 ) ) ;
#13958=DIRECTION ( 'NONE',  ( -0.000000000000000000, -1.000000000000000000, -0.000000000000000000 ) ) ;
#14015=DIRECTION ( 'NONE',  ( 1.000000000000000000, 0.000000000000000000, -0.000000000000000000 ) ) ;
#14048=CARTESIAN_POINT ( 'NONE',  ( 73.69809405469877106, 29.52935533987996664, -27.49288055531513209 ) ) ;
#14084=CARTESIAN_POINT ( 'NONE',  ( 67.21328690825529861, 29.52935533987996664, -21.00807340887166674 ) ) ;
#14153=VERTEX_POINT ( 'NONE', #9664 ) ;
#14243=DIRECTION ( 'NONE',  ( -0.000000000000000000, -0.000000000000000000, -1.000000000000000000 ) ) ;
#14245=APPLICATION_CONTEXT ( 'automotive_design' ) ;
#14271=LINE ( 'NONE', #3719, #6936 ) ;
#14272=ORIENTED_EDGE ( 'NONE', *, *, #2036, .F. ) ;
#14327=VECTOR ( 'NONE', #11685, 1000.000000000000000 ) ;
#14344=FACE_BOUND ( 'NONE', #11914, .T. ) ;
#14352=LINE ( 'NONE', #3796, #9656 ) ;
#14388=ADVANCED_BREP_SHAPE_REPRESENTATION ( '', ( #9491, #6315 ), #10740 ) ;
#14467=CARTESIAN_POINT ( 'NONE',  ( 62.67308791069655882, 25.52935533987996664, -33.00000000000013500 ) ) ;
#14477=CARTESIAN_POINT ( 'NONE',  ( 67.21328690825529861, 29.52935533987996664, -21.00807340887166674 ) ) ;
#14535=ADVANCED_FACE ( 'NONE', ( #390 ), #5086, .T. ) ;
#14541=CARTESIAN_POINT ( 'NONE',  ( 73.69809405469877106, 29.52935533987996664, -21.00807340887166674 ) ) ;
#14612=EDGE_CURVE ( 'NONE', #3738, #791, #9292, .T. ) ;
#14624=ORIENTED_EDGE ( 'NONE', *, *, #1195, .T. ) ;
#14874=CARTESIAN_POINT ( 'NONE',  ( 73.69809405469877106, 29.52935533987996664, -21.00807340887166674 ) ) ;
#14889=DIRECTION ( 'NONE',  ( -0.000000000000000000, -1.000000000000000000, -0.000000000000000000 ) ) ;
#14936=VERTEX_POINT ( 'NONE', #3108 ) ;
#15003=DIRECTION ( 'NONE',  ( 0.000000000000000000, 1.000000000000000000, 0.000000000000000000 ) ) ;
#15006=ADVANCED_FACE ( 'NONE', ( #7735 ), #2104, .F. ) ;
#15048=CARTESIAN_POINT ( 'NONE',  ( 84.72310019870096198, 29.52935533987996664, -33.00000000000013500 ) ) ;
#15088=CARTESIAN_POINT ( 'NONE',  ( 73.69809405469877106, 25.52935533987996664, -21.00807340887166674 ) ) ;
#15120=DIRECTION ( 'NONE',  ( 0.000000000000000000, 0.000000000000000000, 1.000000000000000000 ) ) ;
#15180=AXIS2_PLACEMENT_3D ( 'NONE', #9909, #1734, #13509 ) ;
#15196=AXIS2_PLACEMENT_3D ( 'NONE', #1482, #109, #10533 ) ;
#15227=AXIS2_PLACEMENT_3D ( 'NONE', #12631, #1079, #14015 ) ;
#15252=COLOUR_RGB('Sky Blue',0.24,0.69,0.87);
#15253=FILL_AREA_STYLE_COLOUR('',#15252);
#15254=FILL_AREA_STYLE('',(#15253));
#15255=SURFACE_STYLE_FILL_AREA(#15254);
#15256=SURFACE_SIDE_STYLE('',(#15255));
#15257=SURFACE_STYLE_USAGE(.BOTH.,#15256);
#15258=PRESENTATION_STYLE_ASSIGNMENT((#15257));
ENDSEC;
END-ISO-10303-21;
